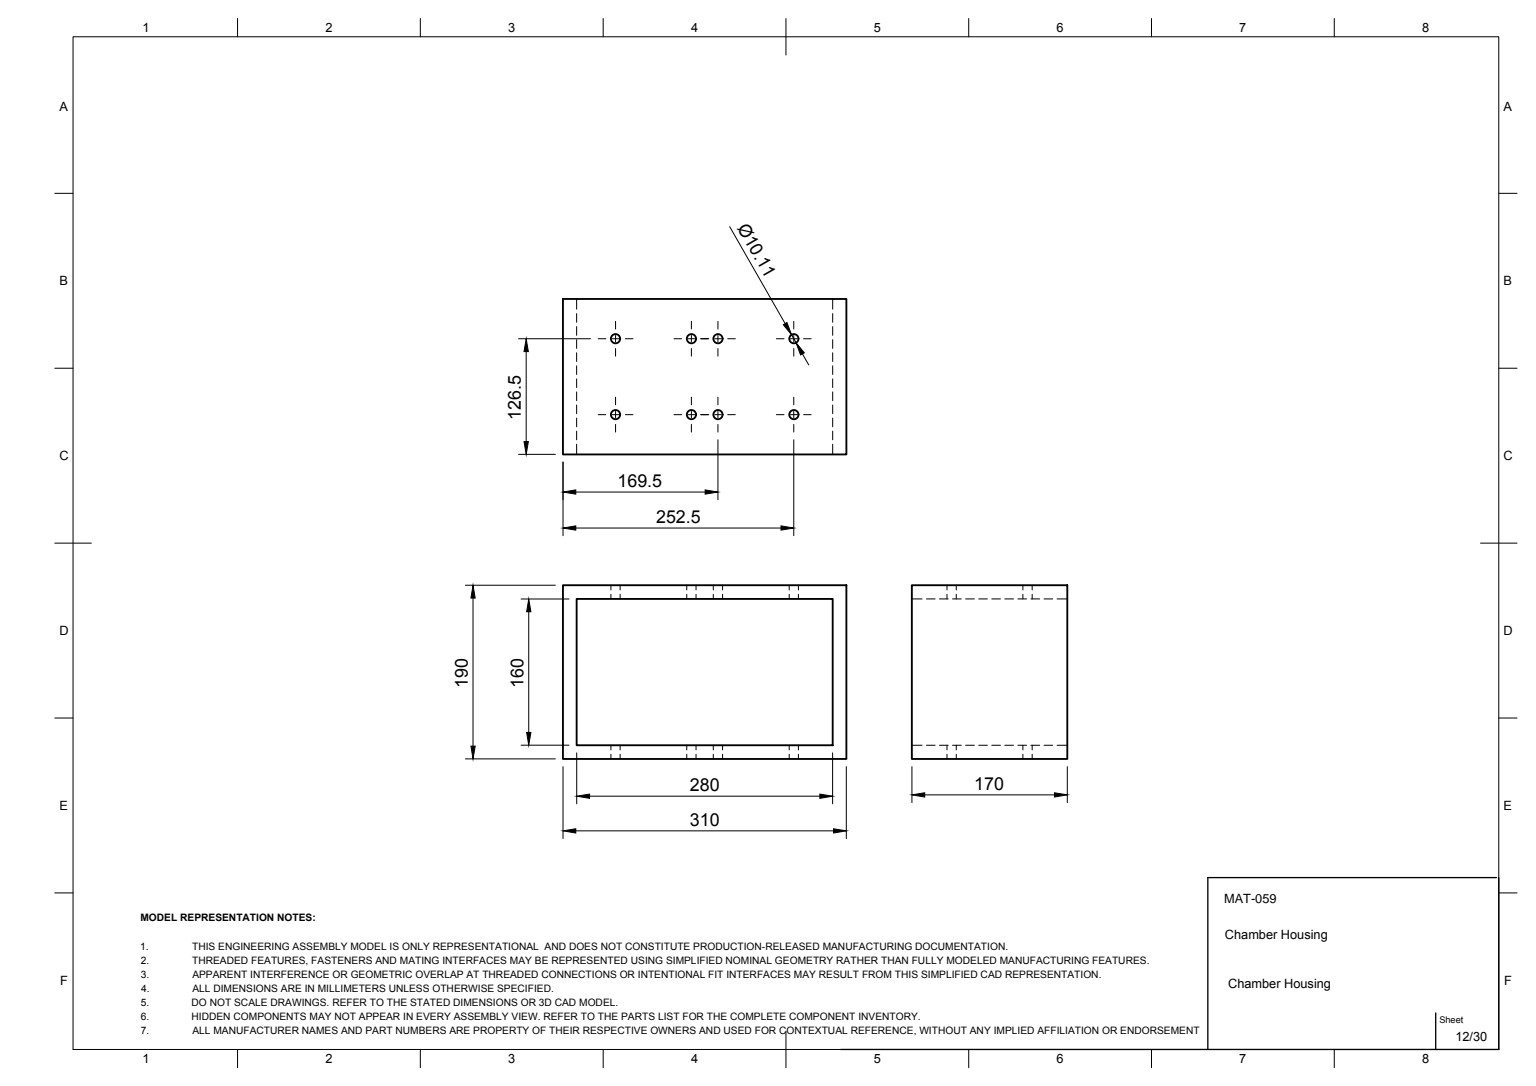
ISO-10303-21;
HEADER;
/* Generated by software containing ST-Developer
 * from STEP Tools, Inc. (www.steptools.com) 
 */

FILE_DESCRIPTION(
/* description */ ('', 'CAx-IF Rec.Pracs.---Representation and Presentation of Product Manufa
cturing Information (PMI)---4.0---2014-10-13'),
/* implementation_level */ '2;1');

FILE_NAME(
/* name */ 'Chamber Housing.step',
/* time_stamp */ '2026-10-28T23:00:48+01:00',
/* author */ (''),
/* organization */ (''),
/* preprocessor_version */ 'ST-DEVELOPER v20.2',
/* originating_system */ 'Autodesk Translation Framework v15.17.0.0',
/* authorisation */ '');

FILE_SCHEMA (('AP242_MANAGED_MODEL_BASED_3D_ENGINEERING_MIM_LF { 1 0 10303 442 2 1 4 }'));
ENDSEC;

DATA;
#10=MECHANICAL_DESIGN_GEOMETRIC_PRESENTATION_REPRESENTATION('',(#986),#61811);
#922=SHAPE_REPRESENTATION_RELATIONSHIP('SRR','None',#61981,#947);
#947=ADVANCED_BREP_SHAPE_REPRESENTATION('',(#1025),#61794);
#986=STYLED_ITEM('',(#62135),#1025);
#1025=MANIFOLD_SOLID_BREP('Body1',#33816);
#1311=CYLINDRICAL_SURFACE('',#35704,5.053);
#1312=CYLINDRICAL_SURFACE('',#35707,5.053);
#1313=CYLINDRICAL_SURFACE('',#35710,5.053);
#1314=CYLINDRICAL_SURFACE('',#35713,5.053);
#1315=CYLINDRICAL_SURFACE('',#35716,5.053);
#1316=CYLINDRICAL_SURFACE('',#35719,5.053);
#1317=CYLINDRICAL_SURFACE('',#35722,5.053);
#1318=CYLINDRICAL_SURFACE('',#35725,5.053);
#1319=CYLINDRICAL_SURFACE('',#35728,5.053);
#1320=CYLINDRICAL_SURFACE('',#35731,5.053);
#1321=CYLINDRICAL_SURFACE('',#35734,5.053);
#1322=CYLINDRICAL_SURFACE('',#35737,5.053);
#1323=CYLINDRICAL_SURFACE('',#35740,5.053);
#1324=CYLINDRICAL_SURFACE('',#35743,5.053);
#1325=CYLINDRICAL_SURFACE('',#35746,5.053);
#1326=CYLINDRICAL_SURFACE('',#35749,5.053);
#2008=FACE_BOUND('',#7101,.T.);
#2009=FACE_BOUND('',#7102,.T.);
#2010=FACE_BOUND('',#7103,.T.);
#2011=FACE_BOUND('',#7104,.T.);
#2012=FACE_BOUND('',#7105,.T.);
#2013=FACE_BOUND('',#7106,.T.);
#2014=FACE_BOUND('',#7107,.T.);
#2015=FACE_BOUND('',#7108,.T.);
#2016=FACE_BOUND('',#7111,.T.);
#2017=FACE_BOUND('',#7112,.T.);
#2018=FACE_BOUND('',#7113,.T.);
#2019=FACE_BOUND('',#7114,.T.);
#2020=FACE_BOUND('',#7115,.T.);
#2021=FACE_BOUND('',#7116,.T.);
#2022=FACE_BOUND('',#7117,.T.);
#2023=FACE_BOUND('',#7118,.T.);
#2024=FACE_BOUND('',#7121,.T.);
#2025=FACE_BOUND('',#7123,.T.);
#2026=FACE_BOUND('',#7124,.T.);
#2027=FACE_BOUND('',#7125,.T.);
#2028=FACE_BOUND('',#7126,.T.);
#2029=FACE_BOUND('',#7127,.T.);
#2030=FACE_BOUND('',#7128,.T.);
#2031=FACE_BOUND('',#7129,.T.);
#2032=FACE_BOUND('',#7130,.T.);
#2033=FACE_BOUND('',#7133,.T.);
#2034=FACE_BOUND('',#7134,.T.);
#2035=FACE_BOUND('',#7135,.T.);
#2036=FACE_BOUND('',#7136,.T.);
#2037=FACE_BOUND('',#7137,.T.);
#2038=FACE_BOUND('',#7138,.T.);
#2039=FACE_BOUND('',#7139,.T.);
#2040=FACE_BOUND('',#7140,.T.);
#2041=FACE_BOUND('',#7143,.T.);
#2920=CIRCLE('',#35705,5.053);
#2921=CIRCLE('',#35706,5.053);
#2922=CIRCLE('',#35708,5.053);
#2923=CIRCLE('',#35709,5.053);
#2924=CIRCLE('',#35711,5.053);
#2925=CIRCLE('',#35712,5.053);
#2926=CIRCLE('',#35714,5.053);
#2927=CIRCLE('',#35715,5.053);
#2928=CIRCLE('',#35717,5.053);
#2929=CIRCLE('',#35718,5.053);
#2930=CIRCLE('',#35720,5.053);
#2931=CIRCLE('',#35721,5.053);
#2932=CIRCLE('',#35723,5.053);
#2933=CIRCLE('',#35724,5.053);
#2934=CIRCLE('',#35726,5.053);
#2935=CIRCLE('',#35727,5.053);
#2936=CIRCLE('',#35729,5.053);
#2937=CIRCLE('',#35730,5.053);
#2938=CIRCLE('',#35732,5.053);
#2939=CIRCLE('',#35733,5.053);
#2940=CIRCLE('',#35735,5.053);
#2941=CIRCLE('',#35736,5.053);
#2942=CIRCLE('',#35738,5.053);
#2943=CIRCLE('',#35739,5.053);
#2944=CIRCLE('',#35741,5.053);
#2945=CIRCLE('',#35742,5.053);
#2946=CIRCLE('',#35744,5.053);
#2947=CIRCLE('',#35745,5.053);
#2948=CIRCLE('',#35747,5.053);
#2949=CIRCLE('',#35748,5.053);
#2950=CIRCLE('',#35750,5.053);
#2951=CIRCLE('',#35751,5.053);
#5076=FACE_OUTER_BOUND('',#7084,.T.);
#5077=FACE_OUTER_BOUND('',#7085,.T.);
#5078=FACE_OUTER_BOUND('',#7086,.T.);
#5079=FACE_OUTER_BOUND('',#7087,.T.);
#5080=FACE_OUTER_BOUND('',#7088,.T.);
#5081=FACE_OUTER_BOUND('',#7089,.T.);
#5082=FACE_OUTER_BOUND('',#7090,.T.);
#5083=FACE_OUTER_BOUND('',#7091,.T.);
#5084=FACE_OUTER_BOUND('',#7092,.T.);
#5085=FACE_OUTER_BOUND('',#7093,.T.);
#5086=FACE_OUTER_BOUND('',#7094,.T.);
#5087=FACE_OUTER_BOUND('',#7095,.T.);
#5088=FACE_OUTER_BOUND('',#7096,.T.);
#5089=FACE_OUTER_BOUND('',#7097,.T.);
#5090=FACE_OUTER_BOUND('',#7098,.T.);
#5091=FACE_OUTER_BOUND('',#7099,.T.);
#5092=FACE_OUTER_BOUND('',#7100,.T.);
#5093=FACE_OUTER_BOUND('',#7109,.T.);
#5094=FACE_OUTER_BOUND('',#7110,.T.);
#5095=FACE_OUTER_BOUND('',#7119,.T.);
#5096=FACE_OUTER_BOUND('',#7120,.T.);
#5097=FACE_OUTER_BOUND('',#7122,.T.);
#5098=FACE_OUTER_BOUND('',#7131,.T.);
#5099=FACE_OUTER_BOUND('',#7132,.T.);
#5100=FACE_OUTER_BOUND('',#7141,.T.);
#5101=FACE_OUTER_BOUND('',#7142,.T.);
#7084=EDGE_LOOP('',(#25654,#25655,#25656,#25657));
#7085=EDGE_LOOP('',(#25658,#25659,#25660,#25661));
#7086=EDGE_LOOP('',(#25662,#25663,#25664,#25665));
#7087=EDGE_LOOP('',(#25666,#25667,#25668,#25669));
#7088=EDGE_LOOP('',(#25670,#25671,#25672,#25673));
#7089=EDGE_LOOP('',(#25674,#25675,#25676,#25677));
#7090=EDGE_LOOP('',(#25678,#25679,#25680,#25681));
#7091=EDGE_LOOP('',(#25682,#25683,#25684,#25685));
#7092=EDGE_LOOP('',(#25686,#25687,#25688,#25689));
#7093=EDGE_LOOP('',(#25690,#25691,#25692,#25693));
#7094=EDGE_LOOP('',(#25694,#25695,#25696,#25697));
#7095=EDGE_LOOP('',(#25698,#25699,#25700,#25701));
#7096=EDGE_LOOP('',(#25702,#25703,#25704,#25705));
#7097=EDGE_LOOP('',(#25706,#25707,#25708,#25709));
#7098=EDGE_LOOP('',(#25710,#25711,#25712,#25713));
#7099=EDGE_LOOP('',(#25714,#25715,#25716,#25717));
#7100=EDGE_LOOP('',(#25718,#25719,#25720,#25721));
#7101=EDGE_LOOP('',(#25722));
#7102=EDGE_LOOP('',(#25723));
#7103=EDGE_LOOP('',(#25724));
#7104=EDGE_LOOP('',(#25725));
#7105=EDGE_LOOP('',(#25726));
#7106=EDGE_LOOP('',(#25727));
#7107=EDGE_LOOP('',(#25728));
#7108=EDGE_LOOP('',(#25729));
#7109=EDGE_LOOP('',(#25730,#25731,#25732,#25733));
#7110=EDGE_LOOP('',(#25734,#25735,#25736,#25737));
#7111=EDGE_LOOP('',(#25738));
#7112=EDGE_LOOP('',(#25739));
#7113=EDGE_LOOP('',(#25740));
#7114=EDGE_LOOP('',(#25741));
#7115=EDGE_LOOP('',(#25742));
#7116=EDGE_LOOP('',(#25743));
#7117=EDGE_LOOP('',(#25744));
#7118=EDGE_LOOP('',(#25745));
#7119=EDGE_LOOP('',(#25746,#25747,#25748,#25749));
#7120=EDGE_LOOP('',(#25750,#25751,#25752,#25753));
#7121=EDGE_LOOP('',(#25754,#25755,#25756,#25757));
#7122=EDGE_LOOP('',(#25758,#25759,#25760,#25761));
#7123=EDGE_LOOP('',(#25762));
#7124=EDGE_LOOP('',(#25763));
#7125=EDGE_LOOP('',(#25764));
#7126=EDGE_LOOP('',(#25765));
#7127=EDGE_LOOP('',(#25766));
#7128=EDGE_LOOP('',(#25767));
#7129=EDGE_LOOP('',(#25768));
#7130=EDGE_LOOP('',(#25769));
#7131=EDGE_LOOP('',(#25770,#25771,#25772,#25773));
#7132=EDGE_LOOP('',(#25774,#25775,#25776,#25777));
#7133=EDGE_LOOP('',(#25778));
#7134=EDGE_LOOP('',(#25779));
#7135=EDGE_LOOP('',(#25780));
#7136=EDGE_LOOP('',(#25781));
#7137=EDGE_LOOP('',(#25782));
#7138=EDGE_LOOP('',(#25783));
#7139=EDGE_LOOP('',(#25784));
#7140=EDGE_LOOP('',(#25785));
#7141=EDGE_LOOP('',(#25786,#25787,#25788,#25789));
#7142=EDGE_LOOP('',(#25790,#25791,#25792,#25793));
#7143=EDGE_LOOP('',(#25794,#25795,#25796,#25797));
#9581=LINE('',#55258,#12128);
#9582=LINE('',#55264,#12129);
#9583=LINE('',#55270,#12130);
#9584=LINE('',#55276,#12131);
#9585=LINE('',#55282,#12132);
#9586=LINE('',#55288,#12133);
#9587=LINE('',#55294,#12134);
#9588=LINE('',#55300,#12135);
#9589=LINE('',#55306,#12136);
#9590=LINE('',#55312,#12137);
#9591=LINE('',#55318,#12138);
#9592=LINE('',#55324,#12139);
#9593=LINE('',#55330,#12140);
#9594=LINE('',#55336,#12141);
#9595=LINE('',#55342,#12142);
#9596=LINE('',#55348,#12143);
#9597=LINE('',#55353,#12144);
#9598=LINE('',#55355,#12145);
#9599=LINE('',#55357,#12146);
#9600=LINE('',#55358,#12147);
#9601=LINE('',#55361,#12148);
#9602=LINE('',#55363,#12149);
#9603=LINE('',#55364,#12150);
#9604=LINE('',#55367,#12151);
#9605=LINE('',#55369,#12152);
#9606=LINE('',#55370,#12153);
#9607=LINE('',#55372,#12154);
#9608=LINE('',#55373,#12155);
#9609=LINE('',#55377,#12156);
#9610=LINE('',#55379,#12157);
#9611=LINE('',#55381,#12158);
#9612=LINE('',#55382,#12159);
#9613=LINE('',#55385,#12160);
#9614=LINE('',#55387,#12161);
#9615=LINE('',#55388,#12162);
#9616=LINE('',#55391,#12163);
#9617=LINE('',#55392,#12164);
#9618=LINE('',#55395,#12165);
#9619=LINE('',#55396,#12166);
#9620=LINE('',#55398,#12167);
#12128=VECTOR('',#42589,5.053);
#12129=VECTOR('',#42596,5.053);
#12130=VECTOR('',#42603,5.053);
#12131=VECTOR('',#42610,5.053);
#12132=VECTOR('',#42617,5.053);
#12133=VECTOR('',#42624,5.053);
#12134=VECTOR('',#42631,5.053);
#12135=VECTOR('',#42638,5.053);
#12136=VECTOR('',#42645,5.053);
#12137=VECTOR('',#42652,5.053);
#12138=VECTOR('',#42659,5.053);
#12139=VECTOR('',#42666,5.053);
#12140=VECTOR('',#42673,5.053);
#12141=VECTOR('',#42680,5.053);
#12142=VECTOR('',#42687,5.053);
#12143=VECTOR('',#42694,5.053);
#12144=VECTOR('',#42699,10.);
#12145=VECTOR('',#42700,10.);
#12146=VECTOR('',#42701,10.);
#12147=VECTOR('',#42702,10.);
#12148=VECTOR('',#42705,10.);
#12149=VECTOR('',#42706,10.);
#12150=VECTOR('',#42707,10.);
#12151=VECTOR('',#42710,10.);
#12152=VECTOR('',#42711,10.);
#12153=VECTOR('',#42712,10.);
#12154=VECTOR('',#42715,10.);
#12155=VECTOR('',#42716,10.);
#12156=VECTOR('',#42719,10.);
#12157=VECTOR('',#42720,10.);
#12158=VECTOR('',#42721,10.);
#12159=VECTOR('',#42722,10.);
#12160=VECTOR('',#42725,10.);
#12161=VECTOR('',#42726,10.);
#12162=VECTOR('',#42727,10.);
#12163=VECTOR('',#42730,10.);
#12164=VECTOR('',#42731,10.);
#12165=VECTOR('',#42734,10.);
#12166=VECTOR('',#42735,10.);
#12167=VECTOR('',#42738,10.);
#14802=VERTEX_POINT('',#55255);
#14803=VERTEX_POINT('',#55257);
#14804=VERTEX_POINT('',#55261);
#14805=VERTEX_POINT('',#55263);
#14806=VERTEX_POINT('',#55267);
#14807=VERTEX_POINT('',#55269);
#14808=VERTEX_POINT('',#55273);
#14809=VERTEX_POINT('',#55275);
#14810=VERTEX_POINT('',#55279);
#14811=VERTEX_POINT('',#55281);
#14812=VERTEX_POINT('',#55285);
#14813=VERTEX_POINT('',#55287);
#14814=VERTEX_POINT('',#55291);
#14815=VERTEX_POINT('',#55293);
#14816=VERTEX_POINT('',#55297);
#14817=VERTEX_POINT('',#55299);
#14818=VERTEX_POINT('',#55303);
#14819=VERTEX_POINT('',#55305);
#14820=VERTEX_POINT('',#55309);
#14821=VERTEX_POINT('',#55311);
#14822=VERTEX_POINT('',#55315);
#14823=VERTEX_POINT('',#55317);
#14824=VERTEX_POINT('',#55321);
#14825=VERTEX_POINT('',#55323);
#14826=VERTEX_POINT('',#55327);
#14827=VERTEX_POINT('',#55329);
#14828=VERTEX_POINT('',#55333);
#14829=VERTEX_POINT('',#55335);
#14830=VERTEX_POINT('',#55339);
#14831=VERTEX_POINT('',#55341);
#14832=VERTEX_POINT('',#55345);
#14833=VERTEX_POINT('',#55347);
#14834=VERTEX_POINT('',#55351);
#14835=VERTEX_POINT('',#55352);
#14836=VERTEX_POINT('',#55354);
#14837=VERTEX_POINT('',#55356);
#14838=VERTEX_POINT('',#55360);
#14839=VERTEX_POINT('',#55362);
#14840=VERTEX_POINT('',#55366);
#14841=VERTEX_POINT('',#55368);
#14842=VERTEX_POINT('',#55375);
#14843=VERTEX_POINT('',#55376);
#14844=VERTEX_POINT('',#55378);
#14845=VERTEX_POINT('',#55380);
#14846=VERTEX_POINT('',#55384);
#14847=VERTEX_POINT('',#55386);
#14848=VERTEX_POINT('',#55390);
#14849=VERTEX_POINT('',#55394);
#18729=EDGE_CURVE('',#14802,#14802,#2920,.T.);
#18730=EDGE_CURVE('',#14802,#14803,#9581,.T.);
#18731=EDGE_CURVE('',#14803,#14803,#2921,.T.);
#18732=EDGE_CURVE('',#14804,#14804,#2922,.T.);
#18733=EDGE_CURVE('',#14804,#14805,#9582,.T.);
#18734=EDGE_CURVE('',#14805,#14805,#2923,.T.);
#18735=EDGE_CURVE('',#14806,#14806,#2924,.T.);
#18736=EDGE_CURVE('',#14806,#14807,#9583,.T.);
#18737=EDGE_CURVE('',#14807,#14807,#2925,.T.);
#18738=EDGE_CURVE('',#14808,#14808,#2926,.T.);
#18739=EDGE_CURVE('',#14808,#14809,#9584,.T.);
#18740=EDGE_CURVE('',#14809,#14809,#2927,.T.);
#18741=EDGE_CURVE('',#14810,#14810,#2928,.T.);
#18742=EDGE_CURVE('',#14810,#14811,#9585,.T.);
#18743=EDGE_CURVE('',#14811,#14811,#2929,.T.);
#18744=EDGE_CURVE('',#14812,#14812,#2930,.T.);
#18745=EDGE_CURVE('',#14812,#14813,#9586,.T.);
#18746=EDGE_CURVE('',#14813,#14813,#2931,.T.);
#18747=EDGE_CURVE('',#14814,#14814,#2932,.T.);
#18748=EDGE_CURVE('',#14814,#14815,#9587,.T.);
#18749=EDGE_CURVE('',#14815,#14815,#2933,.T.);
#18750=EDGE_CURVE('',#14816,#14816,#2934,.T.);
#18751=EDGE_CURVE('',#14816,#14817,#9588,.T.);
#18752=EDGE_CURVE('',#14817,#14817,#2935,.T.);
#18753=EDGE_CURVE('',#14818,#14818,#2936,.T.);
#18754=EDGE_CURVE('',#14818,#14819,#9589,.T.);
#18755=EDGE_CURVE('',#14819,#14819,#2937,.T.);
#18756=EDGE_CURVE('',#14820,#14820,#2938,.T.);
#18757=EDGE_CURVE('',#14820,#14821,#9590,.T.);
#18758=EDGE_CURVE('',#14821,#14821,#2939,.T.);
#18759=EDGE_CURVE('',#14822,#14822,#2940,.T.);
#18760=EDGE_CURVE('',#14822,#14823,#9591,.T.);
#18761=EDGE_CURVE('',#14823,#14823,#2941,.T.);
#18762=EDGE_CURVE('',#14824,#14824,#2942,.T.);
#18763=EDGE_CURVE('',#14824,#14825,#9592,.T.);
#18764=EDGE_CURVE('',#14825,#14825,#2943,.T.);
#18765=EDGE_CURVE('',#14826,#14826,#2944,.T.);
#18766=EDGE_CURVE('',#14826,#14827,#9593,.T.);
#18767=EDGE_CURVE('',#14827,#14827,#2945,.T.);
#18768=EDGE_CURVE('',#14828,#14828,#2946,.T.);
#18769=EDGE_CURVE('',#14828,#14829,#9594,.T.);
#18770=EDGE_CURVE('',#14829,#14829,#2947,.T.);
#18771=EDGE_CURVE('',#14830,#14830,#2948,.T.);
#18772=EDGE_CURVE('',#14830,#14831,#9595,.T.);
#18773=EDGE_CURVE('',#14831,#14831,#2949,.T.);
#18774=EDGE_CURVE('',#14832,#14832,#2950,.T.);
#18775=EDGE_CURVE('',#14832,#14833,#9596,.T.);
#18776=EDGE_CURVE('',#14833,#14833,#2951,.T.);
#18777=EDGE_CURVE('',#14834,#14835,#9597,.T.);
#18778=EDGE_CURVE('',#14836,#14835,#9598,.T.);
#18779=EDGE_CURVE('',#14836,#14837,#9599,.T.);
#18780=EDGE_CURVE('',#14834,#14837,#9600,.T.);
#18781=EDGE_CURVE('',#14838,#14836,#9601,.T.);
#18782=EDGE_CURVE('',#14838,#14839,#9602,.T.);
#18783=EDGE_CURVE('',#14837,#14839,#9603,.T.);
#18784=EDGE_CURVE('',#14840,#14838,#9604,.T.);
#18785=EDGE_CURVE('',#14840,#14841,#9605,.T.);
#18786=EDGE_CURVE('',#14839,#14841,#9606,.T.);
#18787=EDGE_CURVE('',#14835,#14840,#9607,.T.);
#18788=EDGE_CURVE('',#14841,#14834,#9608,.T.);
#18789=EDGE_CURVE('',#14842,#14843,#9609,.T.);
#18790=EDGE_CURVE('',#14843,#14844,#9610,.T.);
#18791=EDGE_CURVE('',#14844,#14845,#9611,.T.);
#18792=EDGE_CURVE('',#14845,#14842,#9612,.T.);
#18793=EDGE_CURVE('',#14846,#14843,#9613,.T.);
#18794=EDGE_CURVE('',#14847,#14846,#9614,.T.);
#18795=EDGE_CURVE('',#14844,#14847,#9615,.T.);
#18796=EDGE_CURVE('',#14848,#14847,#9616,.T.);
#18797=EDGE_CURVE('',#14845,#14848,#9617,.T.);
#18798=EDGE_CURVE('',#14849,#14848,#9618,.T.);
#18799=EDGE_CURVE('',#14842,#14849,#9619,.T.);
#18800=EDGE_CURVE('',#14846,#14849,#9620,.T.);
#25654=ORIENTED_EDGE('',*,*,#18729,.F.);
#25655=ORIENTED_EDGE('',*,*,#18730,.T.);
#25656=ORIENTED_EDGE('',*,*,#18731,.F.);
#25657=ORIENTED_EDGE('',*,*,#18730,.F.);
#25658=ORIENTED_EDGE('',*,*,#18732,.F.);
#25659=ORIENTED_EDGE('',*,*,#18733,.T.);
#25660=ORIENTED_EDGE('',*,*,#18734,.F.);
#25661=ORIENTED_EDGE('',*,*,#18733,.F.);
#25662=ORIENTED_EDGE('',*,*,#18735,.F.);
#25663=ORIENTED_EDGE('',*,*,#18736,.T.);
#25664=ORIENTED_EDGE('',*,*,#18737,.F.);
#25665=ORIENTED_EDGE('',*,*,#18736,.F.);
#25666=ORIENTED_EDGE('',*,*,#18738,.F.);
#25667=ORIENTED_EDGE('',*,*,#18739,.T.);
#25668=ORIENTED_EDGE('',*,*,#18740,.F.);
#25669=ORIENTED_EDGE('',*,*,#18739,.F.);
#25670=ORIENTED_EDGE('',*,*,#18741,.F.);
#25671=ORIENTED_EDGE('',*,*,#18742,.T.);
#25672=ORIENTED_EDGE('',*,*,#18743,.F.);
#25673=ORIENTED_EDGE('',*,*,#18742,.F.);
#25674=ORIENTED_EDGE('',*,*,#18744,.F.);
#25675=ORIENTED_EDGE('',*,*,#18745,.T.);
#25676=ORIENTED_EDGE('',*,*,#18746,.F.);
#25677=ORIENTED_EDGE('',*,*,#18745,.F.);
#25678=ORIENTED_EDGE('',*,*,#18747,.F.);
#25679=ORIENTED_EDGE('',*,*,#18748,.T.);
#25680=ORIENTED_EDGE('',*,*,#18749,.F.);
#25681=ORIENTED_EDGE('',*,*,#18748,.F.);
#25682=ORIENTED_EDGE('',*,*,#18750,.F.);
#25683=ORIENTED_EDGE('',*,*,#18751,.T.);
#25684=ORIENTED_EDGE('',*,*,#18752,.F.);
#25685=ORIENTED_EDGE('',*,*,#18751,.F.);
#25686=ORIENTED_EDGE('',*,*,#18753,.F.);
#25687=ORIENTED_EDGE('',*,*,#18754,.T.);
#25688=ORIENTED_EDGE('',*,*,#18755,.F.);
#25689=ORIENTED_EDGE('',*,*,#18754,.F.);
#25690=ORIENTED_EDGE('',*,*,#18756,.F.);
#25691=ORIENTED_EDGE('',*,*,#18757,.T.);
#25692=ORIENTED_EDGE('',*,*,#18758,.F.);
#25693=ORIENTED_EDGE('',*,*,#18757,.F.);
#25694=ORIENTED_EDGE('',*,*,#18759,.F.);
#25695=ORIENTED_EDGE('',*,*,#18760,.T.);
#25696=ORIENTED_EDGE('',*,*,#18761,.F.);
#25697=ORIENTED_EDGE('',*,*,#18760,.F.);
#25698=ORIENTED_EDGE('',*,*,#18762,.F.);
#25699=ORIENTED_EDGE('',*,*,#18763,.T.);
#25700=ORIENTED_EDGE('',*,*,#18764,.F.);
#25701=ORIENTED_EDGE('',*,*,#18763,.F.);
#25702=ORIENTED_EDGE('',*,*,#18765,.F.);
#25703=ORIENTED_EDGE('',*,*,#18766,.T.);
#25704=ORIENTED_EDGE('',*,*,#18767,.F.);
#25705=ORIENTED_EDGE('',*,*,#18766,.F.);
#25706=ORIENTED_EDGE('',*,*,#18768,.F.);
#25707=ORIENTED_EDGE('',*,*,#18769,.T.);
#25708=ORIENTED_EDGE('',*,*,#18770,.F.);
#25709=ORIENTED_EDGE('',*,*,#18769,.F.);
#25710=ORIENTED_EDGE('',*,*,#18771,.F.);
#25711=ORIENTED_EDGE('',*,*,#18772,.T.);
#25712=ORIENTED_EDGE('',*,*,#18773,.F.);
#25713=ORIENTED_EDGE('',*,*,#18772,.F.);
#25714=ORIENTED_EDGE('',*,*,#18774,.F.);
#25715=ORIENTED_EDGE('',*,*,#18775,.T.);
#25716=ORIENTED_EDGE('',*,*,#18776,.F.);
#25717=ORIENTED_EDGE('',*,*,#18775,.F.);
#25718=ORIENTED_EDGE('',*,*,#18777,.T.);
#25719=ORIENTED_EDGE('',*,*,#18778,.F.);
#25720=ORIENTED_EDGE('',*,*,#18779,.T.);
#25721=ORIENTED_EDGE('',*,*,#18780,.F.);
#25722=ORIENTED_EDGE('',*,*,#18734,.T.);
#25723=ORIENTED_EDGE('',*,*,#18740,.T.);
#25724=ORIENTED_EDGE('',*,*,#18746,.T.);
#25725=ORIENTED_EDGE('',*,*,#18752,.T.);
#25726=ORIENTED_EDGE('',*,*,#18758,.T.);
#25727=ORIENTED_EDGE('',*,*,#18764,.T.);
#25728=ORIENTED_EDGE('',*,*,#18770,.T.);
#25729=ORIENTED_EDGE('',*,*,#18776,.T.);
#25730=ORIENTED_EDGE('',*,*,#18779,.F.);
#25731=ORIENTED_EDGE('',*,*,#18781,.F.);
#25732=ORIENTED_EDGE('',*,*,#18782,.T.);
#25733=ORIENTED_EDGE('',*,*,#18783,.F.);
#25734=ORIENTED_EDGE('',*,*,#18782,.F.);
#25735=ORIENTED_EDGE('',*,*,#18784,.F.);
#25736=ORIENTED_EDGE('',*,*,#18785,.T.);
#25737=ORIENTED_EDGE('',*,*,#18786,.F.);
#25738=ORIENTED_EDGE('',*,*,#18729,.T.);
#25739=ORIENTED_EDGE('',*,*,#18735,.T.);
#25740=ORIENTED_EDGE('',*,*,#18741,.T.);
#25741=ORIENTED_EDGE('',*,*,#18747,.T.);
#25742=ORIENTED_EDGE('',*,*,#18753,.T.);
#25743=ORIENTED_EDGE('',*,*,#18759,.T.);
#25744=ORIENTED_EDGE('',*,*,#18765,.T.);
#25745=ORIENTED_EDGE('',*,*,#18771,.T.);
#25746=ORIENTED_EDGE('',*,*,#18785,.F.);
#25747=ORIENTED_EDGE('',*,*,#18787,.F.);
#25748=ORIENTED_EDGE('',*,*,#18777,.F.);
#25749=ORIENTED_EDGE('',*,*,#18788,.F.);
#25750=ORIENTED_EDGE('',*,*,#18789,.T.);
#25751=ORIENTED_EDGE('',*,*,#18790,.T.);
#25752=ORIENTED_EDGE('',*,*,#18791,.T.);
#25753=ORIENTED_EDGE('',*,*,#18792,.T.);
#25754=ORIENTED_EDGE('',*,*,#18778,.T.);
#25755=ORIENTED_EDGE('',*,*,#18787,.T.);
#25756=ORIENTED_EDGE('',*,*,#18784,.T.);
#25757=ORIENTED_EDGE('',*,*,#18781,.T.);
#25758=ORIENTED_EDGE('',*,*,#18793,.F.);
#25759=ORIENTED_EDGE('',*,*,#18794,.F.);
#25760=ORIENTED_EDGE('',*,*,#18795,.F.);
#25761=ORIENTED_EDGE('',*,*,#18790,.F.);
#25762=ORIENTED_EDGE('',*,*,#18732,.T.);
#25763=ORIENTED_EDGE('',*,*,#18738,.T.);
#25764=ORIENTED_EDGE('',*,*,#18744,.T.);
#25765=ORIENTED_EDGE('',*,*,#18750,.T.);
#25766=ORIENTED_EDGE('',*,*,#18756,.T.);
#25767=ORIENTED_EDGE('',*,*,#18762,.T.);
#25768=ORIENTED_EDGE('',*,*,#18768,.T.);
#25769=ORIENTED_EDGE('',*,*,#18774,.T.);
#25770=ORIENTED_EDGE('',*,*,#18795,.T.);
#25771=ORIENTED_EDGE('',*,*,#18796,.F.);
#25772=ORIENTED_EDGE('',*,*,#18797,.F.);
#25773=ORIENTED_EDGE('',*,*,#18791,.F.);
#25774=ORIENTED_EDGE('',*,*,#18797,.T.);
#25775=ORIENTED_EDGE('',*,*,#18798,.F.);
#25776=ORIENTED_EDGE('',*,*,#18799,.F.);
#25777=ORIENTED_EDGE('',*,*,#18792,.F.);
#25778=ORIENTED_EDGE('',*,*,#18731,.T.);
#25779=ORIENTED_EDGE('',*,*,#18737,.T.);
#25780=ORIENTED_EDGE('',*,*,#18743,.T.);
#25781=ORIENTED_EDGE('',*,*,#18749,.T.);
#25782=ORIENTED_EDGE('',*,*,#18755,.T.);
#25783=ORIENTED_EDGE('',*,*,#18761,.T.);
#25784=ORIENTED_EDGE('',*,*,#18767,.T.);
#25785=ORIENTED_EDGE('',*,*,#18773,.T.);
#25786=ORIENTED_EDGE('',*,*,#18799,.T.);
#25787=ORIENTED_EDGE('',*,*,#18800,.F.);
#25788=ORIENTED_EDGE('',*,*,#18793,.T.);
#25789=ORIENTED_EDGE('',*,*,#18789,.F.);
#25790=ORIENTED_EDGE('',*,*,#18800,.T.);
#25791=ORIENTED_EDGE('',*,*,#18798,.T.);
#25792=ORIENTED_EDGE('',*,*,#18796,.T.);
#25793=ORIENTED_EDGE('',*,*,#18794,.T.);
#25794=ORIENTED_EDGE('',*,*,#18780,.T.);
#25795=ORIENTED_EDGE('',*,*,#18783,.T.);
#25796=ORIENTED_EDGE('',*,*,#18786,.T.);
#25797=ORIENTED_EDGE('',*,*,#18788,.T.);
#31578=PLANE('',#35752);
#31579=PLANE('',#35753);
#31580=PLANE('',#35754);
#31581=PLANE('',#35755);
#31582=PLANE('',#35756);
#31583=PLANE('',#35757);
#31584=PLANE('',#35758);
#31585=PLANE('',#35759);
#31586=PLANE('',#35760);
#31587=PLANE('',#35761);
#32757=ADVANCED_FACE('',(#5076),#1311,.F.);
#32758=ADVANCED_FACE('',(#5077),#1312,.F.);
#32759=ADVANCED_FACE('',(#5078),#1313,.F.);
#32760=ADVANCED_FACE('',(#5079),#1314,.F.);
#32761=ADVANCED_FACE('',(#5080),#1315,.F.);
#32762=ADVANCED_FACE('',(#5081),#1316,.F.);
#32763=ADVANCED_FACE('',(#5082),#1317,.F.);
#32764=ADVANCED_FACE('',(#5083),#1318,.F.);
#32765=ADVANCED_FACE('',(#5084),#1319,.F.);
#32766=ADVANCED_FACE('',(#5085),#1320,.F.);
#32767=ADVANCED_FACE('',(#5086),#1321,.F.);
#32768=ADVANCED_FACE('',(#5087),#1322,.F.);
#32769=ADVANCED_FACE('',(#5088),#1323,.F.);
#32770=ADVANCED_FACE('',(#5089),#1324,.F.);
#32771=ADVANCED_FACE('',(#5090),#1325,.F.);
#32772=ADVANCED_FACE('',(#5091),#1326,.F.);
#32773=ADVANCED_FACE('',(#5092,#2008,#2009,#2010,#2011,#2012,#2013,#2014,
#2015),#31578,.F.);
#32774=ADVANCED_FACE('',(#5093),#31579,.F.);
#32775=ADVANCED_FACE('',(#5094,#2016,#2017,#2018,#2019,#2020,#2021,#2022,
#2023),#31580,.F.);
#32776=ADVANCED_FACE('',(#5095),#31581,.F.);
#32777=ADVANCED_FACE('',(#5096,#2024),#31582,.T.);
#32778=ADVANCED_FACE('',(#5097,#2025,#2026,#2027,#2028,#2029,#2030,#2031,
#2032),#31583,.T.);
#32779=ADVANCED_FACE('',(#5098),#31584,.T.);
#32780=ADVANCED_FACE('',(#5099,#2033,#2034,#2035,#2036,#2037,#2038,#2039,
#2040),#31585,.T.);
#32781=ADVANCED_FACE('',(#5100),#31586,.T.);
#32782=ADVANCED_FACE('',(#5101,#2041),#31587,.T.);
#33816=CLOSED_SHELL('',(#32757,#32758,#32759,#32760,#32761,#32762,#32763,
#32764,#32765,#32766,#32767,#32768,#32769,#32770,#32771,#32772,#32773,#32774,
#32775,#32776,#32777,#32778,#32779,#32780,#32781,#32782));
#35703=AXIS2_PLACEMENT_3D('',#55253,#42583,#42584);
#35704=AXIS2_PLACEMENT_3D('',#55254,#42585,#42586);
#35705=AXIS2_PLACEMENT_3D('',#55256,#42587,#42588);
#35706=AXIS2_PLACEMENT_3D('',#55259,#42590,#42591);
#35707=AXIS2_PLACEMENT_3D('',#55260,#42592,#42593);
#35708=AXIS2_PLACEMENT_3D('',#55262,#42594,#42595);
#35709=AXIS2_PLACEMENT_3D('',#55265,#42597,#42598);
#35710=AXIS2_PLACEMENT_3D('',#55266,#42599,#42600);
#35711=AXIS2_PLACEMENT_3D('',#55268,#42601,#42602);
#35712=AXIS2_PLACEMENT_3D('',#55271,#42604,#42605);
#35713=AXIS2_PLACEMENT_3D('',#55272,#42606,#42607);
#35714=AXIS2_PLACEMENT_3D('',#55274,#42608,#42609);
#35715=AXIS2_PLACEMENT_3D('',#55277,#42611,#42612);
#35716=AXIS2_PLACEMENT_3D('',#55278,#42613,#42614);
#35717=AXIS2_PLACEMENT_3D('',#55280,#42615,#42616);
#35718=AXIS2_PLACEMENT_3D('',#55283,#42618,#42619);
#35719=AXIS2_PLACEMENT_3D('',#55284,#42620,#42621);
#35720=AXIS2_PLACEMENT_3D('',#55286,#42622,#42623);
#35721=AXIS2_PLACEMENT_3D('',#55289,#42625,#42626);
#35722=AXIS2_PLACEMENT_3D('',#55290,#42627,#42628);
#35723=AXIS2_PLACEMENT_3D('',#55292,#42629,#42630);
#35724=AXIS2_PLACEMENT_3D('',#55295,#42632,#42633);
#35725=AXIS2_PLACEMENT_3D('',#55296,#42634,#42635);
#35726=AXIS2_PLACEMENT_3D('',#55298,#42636,#42637);
#35727=AXIS2_PLACEMENT_3D('',#55301,#42639,#42640);
#35728=AXIS2_PLACEMENT_3D('',#55302,#42641,#42642);
#35729=AXIS2_PLACEMENT_3D('',#55304,#42643,#42644);
#35730=AXIS2_PLACEMENT_3D('',#55307,#42646,#42647);
#35731=AXIS2_PLACEMENT_3D('',#55308,#42648,#42649);
#35732=AXIS2_PLACEMENT_3D('',#55310,#42650,#42651);
#35733=AXIS2_PLACEMENT_3D('',#55313,#42653,#42654);
#35734=AXIS2_PLACEMENT_3D('',#55314,#42655,#42656);
#35735=AXIS2_PLACEMENT_3D('',#55316,#42657,#42658);
#35736=AXIS2_PLACEMENT_3D('',#55319,#42660,#42661);
#35737=AXIS2_PLACEMENT_3D('',#55320,#42662,#42663);
#35738=AXIS2_PLACEMENT_3D('',#55322,#42664,#42665);
#35739=AXIS2_PLACEMENT_3D('',#55325,#42667,#42668);
#35740=AXIS2_PLACEMENT_3D('',#55326,#42669,#42670);
#35741=AXIS2_PLACEMENT_3D('',#55328,#42671,#42672);
#35742=AXIS2_PLACEMENT_3D('',#55331,#42674,#42675);
#35743=AXIS2_PLACEMENT_3D('',#55332,#42676,#42677);
#35744=AXIS2_PLACEMENT_3D('',#55334,#42678,#42679);
#35745=AXIS2_PLACEMENT_3D('',#55337,#42681,#42682);
#35746=AXIS2_PLACEMENT_3D('',#55338,#42683,#42684);
#35747=AXIS2_PLACEMENT_3D('',#55340,#42685,#42686);
#35748=AXIS2_PLACEMENT_3D('',#55343,#42688,#42689);
#35749=AXIS2_PLACEMENT_3D('',#55344,#42690,#42691);
#35750=AXIS2_PLACEMENT_3D('',#55346,#42692,#42693);
#35751=AXIS2_PLACEMENT_3D('',#55349,#42695,#42696);
#35752=AXIS2_PLACEMENT_3D('',#55350,#42697,#42698);
#35753=AXIS2_PLACEMENT_3D('',#55359,#42703,#42704);
#35754=AXIS2_PLACEMENT_3D('',#55365,#42708,#42709);
#35755=AXIS2_PLACEMENT_3D('',#55371,#42713,#42714);
#35756=AXIS2_PLACEMENT_3D('',#55374,#42717,#42718);
#35757=AXIS2_PLACEMENT_3D('',#55383,#42723,#42724);
#35758=AXIS2_PLACEMENT_3D('',#55389,#42728,#42729);
#35759=AXIS2_PLACEMENT_3D('',#55393,#42732,#42733);
#35760=AXIS2_PLACEMENT_3D('',#55397,#42736,#42737);
#35761=AXIS2_PLACEMENT_3D('',#55399,#42739,#42740);
#42583=DIRECTION('axis',(0.,0.,1.));
#42584=DIRECTION('refdir',(1.,0.,0.));
#42585=DIRECTION('center_axis',(5.07060489460067E-16,1.,1.05904684225915E-15));
#42586=DIRECTION('ref_axis',(-5.46077161851015E-15,1.05904684225915E-15,
-1.));
#42587=DIRECTION('center_axis',(4.41572679712592E-16,1.,1.05904684225915E-15));
#42588=DIRECTION('ref_axis',(-5.46077161851015E-15,1.05904684225915E-15,
-1.));
#42589=DIRECTION('',(5.07060489460067E-16,1.,1.05904684225915E-15));
#42590=DIRECTION('center_axis',(-5.07060489460067E-16,-1.,-1.05904684225915E-15));
#42591=DIRECTION('ref_axis',(-5.46077161851015E-15,1.05904684225915E-15,
-1.));
#42592=DIRECTION('center_axis',(5.07060489460067E-16,1.,1.05904684225915E-15));
#42593=DIRECTION('ref_axis',(-5.46077161851015E-15,1.05904684225915E-15,
-1.));
#42594=DIRECTION('center_axis',(4.92735031077807E-16,1.,1.05904684225915E-15));
#42595=DIRECTION('ref_axis',(-5.46077161851015E-15,1.05904684225915E-15,
-1.));
#42596=DIRECTION('',(5.07060489460067E-16,1.,1.05904684225915E-15));
#42597=DIRECTION('center_axis',(-4.41572679712592E-16,-1.,-1.05904684225915E-15));
#42598=DIRECTION('ref_axis',(-5.46077161851015E-15,1.05904684225915E-15,
-1.));
#42599=DIRECTION('center_axis',(5.07060489460067E-16,1.,1.05904684225915E-15));
#42600=DIRECTION('ref_axis',(-5.46077161851015E-15,1.05904684225915E-15,
-1.));
#42601=DIRECTION('center_axis',(4.41572679712592E-16,1.,1.05904684225915E-15));
#42602=DIRECTION('ref_axis',(-5.46077161851015E-15,1.05904684225915E-15,
-1.));
#42603=DIRECTION('',(5.07060489460067E-16,1.,1.05904684225915E-15));
#42604=DIRECTION('center_axis',(-5.07060489460067E-16,-1.,-1.05904684225915E-15));
#42605=DIRECTION('ref_axis',(-5.46077161851015E-15,1.05904684225915E-15,
-1.));
#42606=DIRECTION('center_axis',(5.07060489460067E-16,1.,1.05904684225915E-15));
#42607=DIRECTION('ref_axis',(-5.46077161851015E-15,1.05904684225915E-15,
-1.));
#42608=DIRECTION('center_axis',(4.92735031077807E-16,1.,1.05904684225915E-15));
#42609=DIRECTION('ref_axis',(-5.46077161851015E-15,1.05904684225915E-15,
-1.));
#42610=DIRECTION('',(5.07060489460067E-16,1.,1.05904684225915E-15));
#42611=DIRECTION('center_axis',(-4.41572679712592E-16,-1.,-1.05904684225915E-15));
#42612=DIRECTION('ref_axis',(-5.46077161851015E-15,1.05904684225915E-15,
-1.));
#42613=DIRECTION('center_axis',(5.07060489460067E-16,1.,1.05904684225915E-15));
#42614=DIRECTION('ref_axis',(-5.46077161851015E-15,1.05904684225915E-15,
-1.));
#42615=DIRECTION('center_axis',(4.41572679712592E-16,1.,1.05904684225915E-15));
#42616=DIRECTION('ref_axis',(-5.46077161851015E-15,1.05904684225915E-15,
-1.));
#42617=DIRECTION('',(5.07060489460067E-16,1.,1.05904684225915E-15));
#42618=DIRECTION('center_axis',(-5.07060489460067E-16,-1.,-1.05904684225915E-15));
#42619=DIRECTION('ref_axis',(-5.46077161851015E-15,1.05904684225915E-15,
-1.));
#42620=DIRECTION('center_axis',(5.07060489460067E-16,1.,1.05904684225915E-15));
#42621=DIRECTION('ref_axis',(-5.46077161851015E-15,1.05904684225915E-15,
-1.));
#42622=DIRECTION('center_axis',(4.92735031077807E-16,1.,1.05904684225915E-15));
#42623=DIRECTION('ref_axis',(-5.46077161851015E-15,1.05904684225915E-15,
-1.));
#42624=DIRECTION('',(5.07060489460067E-16,1.,1.05904684225915E-15));
#42625=DIRECTION('center_axis',(-4.41572679712592E-16,-1.,-1.05904684225915E-15));
#42626=DIRECTION('ref_axis',(-5.46077161851015E-15,1.05904684225915E-15,
-1.));
#42627=DIRECTION('center_axis',(5.07060489460067E-16,1.,1.05904684225915E-15));
#42628=DIRECTION('ref_axis',(-5.46077161851015E-15,1.05904684225915E-15,
-1.));
#42629=DIRECTION('center_axis',(4.41572679712592E-16,1.,1.05904684225915E-15));
#42630=DIRECTION('ref_axis',(-5.46077161851015E-15,1.05904684225915E-15,
-1.));
#42631=DIRECTION('',(5.07060489460067E-16,1.,1.05904684225915E-15));
#42632=DIRECTION('center_axis',(-5.07060489460067E-16,-1.,-1.05904684225915E-15));
#42633=DIRECTION('ref_axis',(-5.46077161851015E-15,1.05904684225915E-15,
-1.));
#42634=DIRECTION('center_axis',(5.07060489460067E-16,1.,1.05904684225915E-15));
#42635=DIRECTION('ref_axis',(-5.46077161851015E-15,1.05904684225915E-15,
-1.));
#42636=DIRECTION('center_axis',(4.92735031077807E-16,1.,1.05904684225915E-15));
#42637=DIRECTION('ref_axis',(-5.46077161851015E-15,1.05904684225915E-15,
-1.));
#42638=DIRECTION('',(5.07060489460067E-16,1.,1.05904684225915E-15));
#42639=DIRECTION('center_axis',(-4.41572679712592E-16,-1.,-1.05904684225915E-15));
#42640=DIRECTION('ref_axis',(-5.46077161851015E-15,1.05904684225915E-15,
-1.));
#42641=DIRECTION('center_axis',(5.07060489460067E-16,1.,1.05904684225915E-15));
#42642=DIRECTION('ref_axis',(-5.46077161851015E-15,1.05904684225915E-15,
-1.));
#42643=DIRECTION('center_axis',(4.41572679712592E-16,1.,1.05904684225915E-15));
#42644=DIRECTION('ref_axis',(-5.46077161851015E-15,1.05904684225915E-15,
-1.));
#42645=DIRECTION('',(5.07060489460067E-16,1.,1.05904684225915E-15));
#42646=DIRECTION('center_axis',(-5.07060489460067E-16,-1.,-1.05904684225915E-15));
#42647=DIRECTION('ref_axis',(-5.46077161851015E-15,1.05904684225915E-15,
-1.));
#42648=DIRECTION('center_axis',(5.07060489460067E-16,1.,1.05904684225915E-15));
#42649=DIRECTION('ref_axis',(-5.46077161851015E-15,1.05904684225915E-15,
-1.));
#42650=DIRECTION('center_axis',(4.92735031077807E-16,1.,1.05904684225915E-15));
#42651=DIRECTION('ref_axis',(-5.46077161851015E-15,1.05904684225915E-15,
-1.));
#42652=DIRECTION('',(5.07060489460067E-16,1.,1.05904684225915E-15));
#42653=DIRECTION('center_axis',(-4.41572679712592E-16,-1.,-1.05904684225915E-15));
#42654=DIRECTION('ref_axis',(-5.46077161851015E-15,1.05904684225915E-15,
-1.));
#42655=DIRECTION('center_axis',(5.07060489460067E-16,1.,1.05904684225915E-15));
#42656=DIRECTION('ref_axis',(-5.46077161851015E-15,1.05904684225915E-15,
-1.));
#42657=DIRECTION('center_axis',(4.41572679712592E-16,1.,1.05904684225915E-15));
#42658=DIRECTION('ref_axis',(-5.46077161851015E-15,1.05904684225915E-15,
-1.));
#42659=DIRECTION('',(5.07060489460067E-16,1.,1.05904684225915E-15));
#42660=DIRECTION('center_axis',(-5.07060489460067E-16,-1.,-1.05904684225915E-15));
#42661=DIRECTION('ref_axis',(-5.46077161851015E-15,1.05904684225915E-15,
-1.));
#42662=DIRECTION('center_axis',(5.07060489460067E-16,1.,1.05904684225915E-15));
#42663=DIRECTION('ref_axis',(-5.46077161851015E-15,1.05904684225915E-15,
-1.));
#42664=DIRECTION('center_axis',(4.92735031077807E-16,1.,1.05904684225915E-15));
#42665=DIRECTION('ref_axis',(-5.46077161851015E-15,1.05904684225915E-15,
-1.));
#42666=DIRECTION('',(5.07060489460067E-16,1.,1.05904684225915E-15));
#42667=DIRECTION('center_axis',(-4.41572679712592E-16,-1.,-1.05904684225915E-15));
#42668=DIRECTION('ref_axis',(-5.46077161851015E-15,1.05904684225915E-15,
-1.));
#42669=DIRECTION('center_axis',(5.07060489460067E-16,1.,1.05904684225915E-15));
#42670=DIRECTION('ref_axis',(-5.46077161851015E-15,1.05904684225915E-15,
-1.));
#42671=DIRECTION('center_axis',(4.41572679712592E-16,1.,1.05904684225915E-15));
#42672=DIRECTION('ref_axis',(-5.46077161851015E-15,1.05904684225915E-15,
-1.));
#42673=DIRECTION('',(5.07060489460067E-16,1.,1.05904684225915E-15));
#42674=DIRECTION('center_axis',(-5.07060489460067E-16,-1.,-1.05904684225915E-15));
#42675=DIRECTION('ref_axis',(-5.46077161851015E-15,1.05904684225915E-15,
-1.));
#42676=DIRECTION('center_axis',(5.07060489460067E-16,1.,1.05904684225915E-15));
#42677=DIRECTION('ref_axis',(-5.46077161851015E-15,1.05904684225915E-15,
-1.));
#42678=DIRECTION('center_axis',(4.92735031077807E-16,1.,1.05904684225915E-15));
#42679=DIRECTION('ref_axis',(-5.46077161851015E-15,1.05904684225915E-15,
-1.));
#42680=DIRECTION('',(5.07060489460067E-16,1.,1.05904684225915E-15));
#42681=DIRECTION('center_axis',(-4.41572679712592E-16,-1.,-1.05904684225915E-15));
#42682=DIRECTION('ref_axis',(-5.46077161851015E-15,1.05904684225915E-15,
-1.));
#42683=DIRECTION('center_axis',(5.07060489460067E-16,1.,1.05904684225915E-15));
#42684=DIRECTION('ref_axis',(-5.46077161851015E-15,1.05904684225915E-15,
-1.));
#42685=DIRECTION('center_axis',(4.41572679712592E-16,1.,1.05904684225915E-15));
#42686=DIRECTION('ref_axis',(-5.46077161851015E-15,1.05904684225915E-15,
-1.));
#42687=DIRECTION('',(5.07060489460067E-16,1.,1.05904684225915E-15));
#42688=DIRECTION('center_axis',(-5.07060489460067E-16,-1.,-1.05904684225915E-15));
#42689=DIRECTION('ref_axis',(-5.46077161851015E-15,1.05904684225915E-15,
-1.));
#42690=DIRECTION('center_axis',(5.07060489460067E-16,1.,1.05904684225915E-15));
#42691=DIRECTION('ref_axis',(-5.46077161851015E-15,1.05904684225915E-15,
-1.));
#42692=DIRECTION('center_axis',(4.92735031077807E-16,1.,1.05904684225915E-15));
#42693=DIRECTION('ref_axis',(-5.46077161851015E-15,1.05904684225915E-15,
-1.));
#42694=DIRECTION('',(5.07060489460067E-16,1.,1.05904684225915E-15));
#42695=DIRECTION('center_axis',(-4.41572679712592E-16,-1.,-1.05904684225915E-15));
#42696=DIRECTION('ref_axis',(-5.46077161851015E-15,1.05904684225915E-15,
-1.));
#42697=DIRECTION('center_axis',(-4.41572679712592E-16,-1.,-1.05904684225915E-15));
#42698=DIRECTION('ref_axis',(-1.,4.41572679712586E-16,5.46077161851015E-15));
#42699=DIRECTION('',(5.46077161851015E-15,-1.05904684225915E-15,1.));
#42700=DIRECTION('',(-1.,4.41572679712586E-16,5.46077161851015E-15));
#42701=DIRECTION('',(-5.46077161851015E-15,1.05904684225915E-15,-1.));
#42702=DIRECTION('',(1.,-4.41572679712586E-16,-5.46077161851015E-15));
#42703=DIRECTION('center_axis',(1.,-3.7813136401972E-16,-5.46077161851015E-15));
#42704=DIRECTION('ref_axis',(-3.78131364019726E-16,-1.,-1.05904684225915E-15));
#42705=DIRECTION('',(-3.78131364019726E-16,-1.,-1.05904684225915E-15));
#42706=DIRECTION('',(-5.46077161851015E-15,1.05904684225915E-15,-1.));
#42707=DIRECTION('',(3.78131364019726E-16,1.,1.05904684225915E-15));
#42708=DIRECTION('center_axis',(4.41572679712592E-16,1.,1.05904684225915E-15));
#42709=DIRECTION('ref_axis',(1.,-4.41572679712586E-16,-5.46077161851015E-15));
#42710=DIRECTION('',(1.,-4.41572679712586E-16,-5.46077161851015E-15));
#42711=DIRECTION('',(-5.46077161851015E-15,1.05904684225915E-15,-1.));
#42712=DIRECTION('',(-1.,4.41572679712586E-16,5.46077161851015E-15));
#42713=DIRECTION('center_axis',(-1.,3.7813136401972E-16,5.46077161851015E-15));
#42714=DIRECTION('ref_axis',(3.78131364019726E-16,1.,1.05904684225915E-15));
#42715=DIRECTION('',(3.78131364019726E-16,1.,1.05904684225915E-15));
#42716=DIRECTION('',(-3.78131364019726E-16,-1.,-1.05904684225915E-15));
#42717=DIRECTION('center_axis',(5.46077161851015E-15,-1.05904684225915E-15,
1.));
#42718=DIRECTION('ref_axis',(3.78131364019726E-16,1.,1.05904684225915E-15));
#42719=DIRECTION('',(-3.78131364019726E-16,-1.,-1.05904684225915E-15));
#42720=DIRECTION('',(1.,-4.92735031077801E-16,-5.46077161851015E-15));
#42721=DIRECTION('',(5.6511629448291E-16,1.,1.05904684225915E-15));
#42722=DIRECTION('',(-1.,5.07060489460061E-16,5.46077161851015E-15));
#42723=DIRECTION('center_axis',(-4.92735031077807E-16,-1.,-1.05904684225915E-15));
#42724=DIRECTION('ref_axis',(-1.,4.92735031077801E-16,5.46077161851015E-15));
#42725=DIRECTION('',(5.46077161851015E-15,-1.05904684225915E-15,1.));
#42726=DIRECTION('',(-1.,4.92735031077801E-16,5.46077161851015E-15));
#42727=DIRECTION('',(-5.46077161851015E-15,1.05904684225915E-15,-1.));
#42728=DIRECTION('center_axis',(1.,-5.65116294482904E-16,-5.46077161851015E-15));
#42729=DIRECTION('ref_axis',(-5.6511629448291E-16,-1.,-1.05904684225915E-15));
#42730=DIRECTION('',(-5.6511629448291E-16,-1.,-1.05904684225915E-15));
#42731=DIRECTION('',(-5.46077161851015E-15,1.05904684225915E-15,-1.));
#42732=DIRECTION('center_axis',(5.07060489460067E-16,1.,1.05904684225915E-15));
#42733=DIRECTION('ref_axis',(1.,-5.07060489460061E-16,-5.46077161851015E-15));
#42734=DIRECTION('',(1.,-5.07060489460061E-16,-5.46077161851015E-15));
#42735=DIRECTION('',(-5.46077161851015E-15,1.05904684225915E-15,-1.));
#42736=DIRECTION('center_axis',(-1.,3.7813136401972E-16,5.46077161851015E-15));
#42737=DIRECTION('ref_axis',(3.78131364019726E-16,1.,1.05904684225915E-15));
#42738=DIRECTION('',(3.78131364019726E-16,1.,1.05904684225915E-15));
#42739=DIRECTION('center_axis',(-5.46077161851015E-15,1.05904684225915E-15,
-1.));
#42740=DIRECTION('ref_axis',(-3.78131364019726E-16,-1.,-1.05904684225915E-15));
#55253=CARTESIAN_POINT('',(0.,0.,0.));
#55254=CARTESIAN_POINT('Origin',(221.615917770968,-486.84465207658,486.500000551893));
#55255=CARTESIAN_POINT('',(221.615917770968,-100.47200726879,491.553000551893));
#55256=CARTESIAN_POINT('Origin',(221.615917770968,-100.47200726879,486.500000551893));
#55257=CARTESIAN_POINT('',(221.615917770968,-85.47200726879,491.553000551893));
#55258=CARTESIAN_POINT('',(221.615917770968,-486.84465207658,491.553000551893));
#55259=CARTESIAN_POINT('Origin',(221.615917770968,-85.47200726879,486.500000551893));
#55260=CARTESIAN_POINT('Origin',(221.615917770968,-486.84465207658,486.500000551893));
#55261=CARTESIAN_POINT('',(221.615917770968,-275.47200726879,491.553000551893));
#55262=CARTESIAN_POINT('Origin',(221.615917770968,-275.47200726879,486.500000551893));
#55263=CARTESIAN_POINT('',(221.615917770968,-260.47200726879,491.553000551893));
#55264=CARTESIAN_POINT('',(221.615917770968,-486.84465207658,491.553000551893));
#55265=CARTESIAN_POINT('Origin',(221.615917770968,-260.47200726879,486.500000551893));
#55266=CARTESIAN_POINT('Origin',(304.615917770968,-486.84465207658,403.500000551892));
#55267=CARTESIAN_POINT('',(304.615917770968,-100.47200726879,408.553000551893));
#55268=CARTESIAN_POINT('Origin',(304.615917770968,-100.47200726879,403.500000551893));
#55269=CARTESIAN_POINT('',(304.615917770968,-85.47200726879,408.553000551893));
#55270=CARTESIAN_POINT('',(304.615917770968,-486.84465207658,408.553000551892));
#55271=CARTESIAN_POINT('Origin',(304.615917770968,-85.47200726879,403.500000551893));
#55272=CARTESIAN_POINT('Origin',(304.615917770968,-486.84465207658,403.500000551892));
#55273=CARTESIAN_POINT('',(304.615917770968,-275.47200726879,408.553000551893));
#55274=CARTESIAN_POINT('Origin',(304.615917770968,-275.47200726879,403.500000551893));
#55275=CARTESIAN_POINT('',(304.615917770968,-260.47200726879,408.553000551893));
#55276=CARTESIAN_POINT('',(304.615917770968,-486.84465207658,408.553000551892));
#55277=CARTESIAN_POINT('Origin',(304.615917770968,-260.47200726879,403.500000551893));
#55278=CARTESIAN_POINT('Origin',(333.615917770968,-486.84465207658,486.500000551892));
#55279=CARTESIAN_POINT('',(333.615917770968,-100.47200726879,491.553000551893));
#55280=CARTESIAN_POINT('Origin',(333.615917770968,-100.47200726879,486.500000551893));
#55281=CARTESIAN_POINT('',(333.615917770969,-85.47200726879,491.553000551893));
#55282=CARTESIAN_POINT('',(333.615917770968,-486.84465207658,491.553000551892));
#55283=CARTESIAN_POINT('Origin',(333.615917770968,-85.4720072687901,486.500000551893));
#55284=CARTESIAN_POINT('Origin',(333.615917770968,-486.84465207658,486.500000551892));
#55285=CARTESIAN_POINT('',(333.615917770968,-275.47200726879,491.553000551893));
#55286=CARTESIAN_POINT('Origin',(333.615917770968,-275.47200726879,486.500000551893));
#55287=CARTESIAN_POINT('',(333.615917770968,-260.47200726879,491.553000551893));
#55288=CARTESIAN_POINT('',(333.615917770968,-486.84465207658,491.553000551892));
#55289=CARTESIAN_POINT('Origin',(333.615917770968,-260.47200726879,486.500000551893));
#55290=CARTESIAN_POINT('Origin',(416.615917770968,-486.84465207658,403.500000551892));
#55291=CARTESIAN_POINT('',(416.615917770968,-100.47200726879,408.553000551892));
#55292=CARTESIAN_POINT('Origin',(416.615917770968,-100.47200726879,403.500000551892));
#55293=CARTESIAN_POINT('',(416.615917770968,-85.4720072687901,408.553000551892));
#55294=CARTESIAN_POINT('',(416.615917770968,-486.84465207658,408.553000551892));
#55295=CARTESIAN_POINT('Origin',(416.615917770968,-85.47200726879,403.500000551892));
#55296=CARTESIAN_POINT('Origin',(416.615917770968,-486.84465207658,403.500000551892));
#55297=CARTESIAN_POINT('',(416.615917770968,-275.47200726879,408.553000551892));
#55298=CARTESIAN_POINT('Origin',(416.615917770968,-275.47200726879,403.500000551892));
#55299=CARTESIAN_POINT('',(416.615917770968,-260.47200726879,408.553000551892));
#55300=CARTESIAN_POINT('',(416.615917770968,-486.84465207658,408.553000551892));
#55301=CARTESIAN_POINT('Origin',(416.615917770968,-260.47200726879,403.500000551892));
#55302=CARTESIAN_POINT('Origin',(333.615917770968,-486.84465207658,403.500000551892));
#55303=CARTESIAN_POINT('',(333.615917770968,-100.47200726879,408.553000551893));
#55304=CARTESIAN_POINT('Origin',(333.615917770968,-100.47200726879,403.500000551893));
#55305=CARTESIAN_POINT('',(333.615917770968,-85.47200726879,408.553000551893));
#55306=CARTESIAN_POINT('',(333.615917770968,-486.84465207658,408.553000551892));
#55307=CARTESIAN_POINT('Origin',(333.615917770968,-85.47200726879,403.500000551893));
#55308=CARTESIAN_POINT('Origin',(333.615917770968,-486.84465207658,403.500000551892));
#55309=CARTESIAN_POINT('',(333.615917770968,-275.47200726879,408.553000551893));
#55310=CARTESIAN_POINT('Origin',(333.615917770968,-275.47200726879,403.500000551893));
#55311=CARTESIAN_POINT('',(333.615917770968,-260.47200726879,408.553000551893));
#55312=CARTESIAN_POINT('',(333.615917770968,-486.84465207658,408.553000551892));
#55313=CARTESIAN_POINT('Origin',(333.615917770968,-260.47200726879,403.500000551893));
#55314=CARTESIAN_POINT('Origin',(416.615917770968,-486.84465207658,486.500000551892));
#55315=CARTESIAN_POINT('',(416.615917770968,-100.47200726879,491.553000551892));
#55316=CARTESIAN_POINT('Origin',(416.615917770968,-100.47200726879,486.500000551892));
#55317=CARTESIAN_POINT('',(416.615917770968,-85.4720072687901,491.553000551892));
#55318=CARTESIAN_POINT('',(416.615917770968,-486.84465207658,491.553000551892));
#55319=CARTESIAN_POINT('Origin',(416.615917770968,-85.4720072687901,486.500000551892));
#55320=CARTESIAN_POINT('Origin',(416.615917770968,-486.84465207658,486.500000551892));
#55321=CARTESIAN_POINT('',(416.615917770968,-275.47200726879,491.553000551892));
#55322=CARTESIAN_POINT('Origin',(416.615917770968,-275.47200726879,486.500000551892));
#55323=CARTESIAN_POINT('',(416.615917770968,-260.47200726879,491.553000551892));
#55324=CARTESIAN_POINT('',(416.615917770968,-486.84465207658,491.553000551892));
#55325=CARTESIAN_POINT('Origin',(416.615917770968,-260.47200726879,486.500000551892));
#55326=CARTESIAN_POINT('Origin',(304.615917770968,-486.84465207658,486.500000551892));
#55327=CARTESIAN_POINT('',(304.615917770968,-100.47200726879,491.553000551893));
#55328=CARTESIAN_POINT('Origin',(304.615917770968,-100.47200726879,486.500000551893));
#55329=CARTESIAN_POINT('',(304.615917770968,-85.47200726879,491.553000551893));
#55330=CARTESIAN_POINT('',(304.615917770968,-486.84465207658,491.553000551892));
#55331=CARTESIAN_POINT('Origin',(304.615917770968,-85.4720072687901,486.500000551893));
#55332=CARTESIAN_POINT('Origin',(304.615917770968,-486.84465207658,486.500000551892));
#55333=CARTESIAN_POINT('',(304.615917770968,-275.47200726879,491.553000551893));
#55334=CARTESIAN_POINT('Origin',(304.615917770968,-275.47200726879,486.500000551893));
#55335=CARTESIAN_POINT('',(304.615917770968,-260.47200726879,491.553000551893));
#55336=CARTESIAN_POINT('',(304.615917770968,-486.84465207658,491.553000551892));
#55337=CARTESIAN_POINT('Origin',(304.615917770968,-260.47200726879,486.500000551893));
#55338=CARTESIAN_POINT('Origin',(221.615917770968,-486.84465207658,403.500000551893));
#55339=CARTESIAN_POINT('',(221.615917770968,-100.47200726879,408.553000551893));
#55340=CARTESIAN_POINT('Origin',(221.615917770968,-100.47200726879,403.500000551893));
#55341=CARTESIAN_POINT('',(221.615917770968,-85.47200726879,408.553000551893));
#55342=CARTESIAN_POINT('',(221.615917770968,-486.84465207658,408.553000551893));
#55343=CARTESIAN_POINT('Origin',(221.615917770968,-85.47200726879,403.500000551893));
#55344=CARTESIAN_POINT('Origin',(221.615917770968,-486.84465207658,403.500000551893));
#55345=CARTESIAN_POINT('',(221.615917770968,-275.47200726879,408.553000551893));
#55346=CARTESIAN_POINT('Origin',(221.615917770968,-275.47200726879,403.500000551893));
#55347=CARTESIAN_POINT('',(221.615917770968,-260.47200726879,408.553000551893));
#55348=CARTESIAN_POINT('',(221.615917770968,-486.84465207658,408.553000551893));
#55349=CARTESIAN_POINT('Origin',(221.615917770968,-260.47200726879,403.500000551893));
#55350=CARTESIAN_POINT('Origin',(459.115917770997,-260.47200726879,445.000000551892));
#55351=CARTESIAN_POINT('',(179.115917770997,-260.47200726879,360.000000551893));
#55352=CARTESIAN_POINT('',(179.115917770997,-260.47200726879,530.000000551893));
#55353=CARTESIAN_POINT('',(179.115917770997,-260.47200726879,445.000000551893));
#55354=CARTESIAN_POINT('',(459.115917770997,-260.47200726879,530.000000551892));
#55355=CARTESIAN_POINT('',(389.115917770983,-260.47200726879,530.000000551892));
#55356=CARTESIAN_POINT('',(459.115917770997,-260.47200726879,360.000000551892));
#55357=CARTESIAN_POINT('',(459.115917770997,-260.47200726879,445.000000551892));
#55358=CARTESIAN_POINT('',(389.115917770982,-260.47200726879,360.000000551892));
#55359=CARTESIAN_POINT('Origin',(459.115917770997,-100.47200726879,445.000000551892));
#55360=CARTESIAN_POINT('',(459.115917770997,-100.47200726879,530.000000551892));
#55361=CARTESIAN_POINT('',(459.115917770997,-140.47200726879,530.000000551892));
#55362=CARTESIAN_POINT('',(459.115917770997,-100.47200726879,360.000000551892));
#55363=CARTESIAN_POINT('',(459.115917770997,-100.47200726879,445.000000551892));
#55364=CARTESIAN_POINT('',(459.115917770997,-140.47200726879,360.000000551892));
#55365=CARTESIAN_POINT('Origin',(179.115917770997,-100.47200726879,445.000000551894));
#55366=CARTESIAN_POINT('',(179.115917770997,-100.47200726879,530.000000551894));
#55367=CARTESIAN_POINT('',(249.115917770983,-100.47200726879,530.000000551893));
#55368=CARTESIAN_POINT('',(179.115917770997,-100.47200726879,360.000000551894));
#55369=CARTESIAN_POINT('',(179.115917770997,-100.47200726879,445.000000551894));
#55370=CARTESIAN_POINT('',(249.115917770982,-100.47200726879,360.000000551893));
#55371=CARTESIAN_POINT('Origin',(179.115917770997,-260.47200726879,445.000000551893));
#55372=CARTESIAN_POINT('',(179.115917770997,-220.47200726879,530.000000551893));
#55373=CARTESIAN_POINT('',(179.115917770997,-220.47200726879,360.000000551893));
#55374=CARTESIAN_POINT('Origin',(319.115917770969,-180.47200726879,530.000000551893));
#55375=CARTESIAN_POINT('',(164.115917770969,-85.4720072687901,530.000000551894));
#55376=CARTESIAN_POINT('',(164.115917770969,-275.47200726879,530.000000551893));
#55377=CARTESIAN_POINT('',(164.115917770969,-275.47200726879,530.000000551893));
#55378=CARTESIAN_POINT('',(474.115917770968,-275.47200726879,530.000000551892));
#55379=CARTESIAN_POINT('',(474.115917770968,-275.47200726879,530.000000551892));
#55380=CARTESIAN_POINT('',(474.115917770969,-85.4720072687902,530.000000551892));
#55381=CARTESIAN_POINT('',(474.115917770969,-85.4720072687902,530.000000551892));
#55382=CARTESIAN_POINT('',(164.115917770969,-85.4720072687901,530.000000551894));
#55383=CARTESIAN_POINT('Origin',(474.115917770968,-275.47200726879,445.000000551892));
#55384=CARTESIAN_POINT('',(164.115917770968,-275.47200726879,360.000000551893));
#55385=CARTESIAN_POINT('',(164.115917770968,-275.47200726879,445.000000551893));
#55386=CARTESIAN_POINT('',(474.115917770968,-275.47200726879,360.000000551892));
#55387=CARTESIAN_POINT('',(474.115917770968,-275.47200726879,360.000000551892));
#55388=CARTESIAN_POINT('',(474.115917770968,-275.47200726879,445.000000551892));
#55389=CARTESIAN_POINT('Origin',(474.115917770968,-85.4720072687901,445.000000551892));
#55390=CARTESIAN_POINT('',(474.115917770968,-85.47200726879,360.000000551892));
#55391=CARTESIAN_POINT('',(474.115917770968,-85.47200726879,360.000000551892));
#55392=CARTESIAN_POINT('',(474.115917770968,-85.4720072687901,445.000000551892));
#55393=CARTESIAN_POINT('Origin',(164.115917770968,-85.47200726879,445.000000551894));
#55394=CARTESIAN_POINT('',(164.115917770968,-85.4720072687899,360.000000551894));
#55395=CARTESIAN_POINT('',(164.115917770968,-85.4720072687899,360.000000551894));
#55396=CARTESIAN_POINT('',(164.115917770968,-85.47200726879,445.000000551894));
#55397=CARTESIAN_POINT('Origin',(164.115917770968,-275.47200726879,445.000000551893));
#55398=CARTESIAN_POINT('',(164.115917770968,-275.47200726879,360.000000551893));
#55399=CARTESIAN_POINT('Origin',(319.115917770968,-180.47200726879,360.000000551893));
#61763=UNCERTAINTY_MEASURE_WITH_UNIT(LENGTH_MEASURE(0.01),#61812,
'DISTANCE_ACCURACY_VALUE',
'Maximum model space distance between geometric entities at asserted c
onnectivities');
#61780=UNCERTAINTY_MEASURE_WITH_UNIT(LENGTH_MEASURE(0.01),#61812,
'DISTANCE_ACCURACY_VALUE',
'Maximum model space distance between geometric entities at asserted c
onnectivities');
#61794=(
GEOMETRIC_REPRESENTATION_CONTEXT(3)
GLOBAL_UNCERTAINTY_ASSIGNED_CONTEXT((#61763))
GLOBAL_UNIT_ASSIGNED_CONTEXT((#61812,#61814,#61815))
REPRESENTATION_CONTEXT('','3D')
);
#61811=(
GEOMETRIC_REPRESENTATION_CONTEXT(3)
GLOBAL_UNCERTAINTY_ASSIGNED_CONTEXT((#61780))
GLOBAL_UNIT_ASSIGNED_CONTEXT((#61812,#61814,#61815))
REPRESENTATION_CONTEXT('','3D')
);
#61812=(
LENGTH_UNIT()
NAMED_UNIT(*)
SI_UNIT(.MILLI.,.METRE.)
);
#61814=(
NAMED_UNIT(*)
PLANE_ANGLE_UNIT()
SI_UNIT($,.RADIAN.)
);
#61815=(
NAMED_UNIT(*)
SI_UNIT($,.STERADIAN.)
SOLID_ANGLE_UNIT()
);
#61829=SHAPE_DEFINITION_REPRESENTATION(#61859,#61981);
#61859=PRODUCT_DEFINITION_SHAPE('',$,#62012);
#61981=SHAPE_REPRESENTATION('',(#35703),#61794);
#61998=PRODUCT_DEFINITION_CONTEXT('part definition',#62090,'design');
#62012=PRODUCT_DEFINITION('Chamber Housing','Chamber Housing',#62042,#61998);
#62042=PRODUCT_DEFINITION_FORMATION('',$,#62105);
#62090=APPLICATION_CONTEXT('Managed model based 3d engineering');
#62091=PRODUCT_CONTEXT('part definition',#62090,'mechanical');
#62105=PRODUCT('Chamber Housing','Chamber Housing',$,(#62091));
#62129=COLOUR_RGB('Dark Blue',0.08,0.2,0.34);
#62130=FILL_AREA_STYLE_COLOUR('',#62129);
#62131=FILL_AREA_STYLE('',(#62130));
#62132=SURFACE_STYLE_FILL_AREA(#62131);
#62133=SURFACE_SIDE_STYLE('',(#62132));
#62134=SURFACE_STYLE_USAGE(.BOTH.,#62133);
#62135=PRESENTATION_STYLE_ASSIGNMENT((#62134));
ENDSEC;
END-ISO-10303-21;
